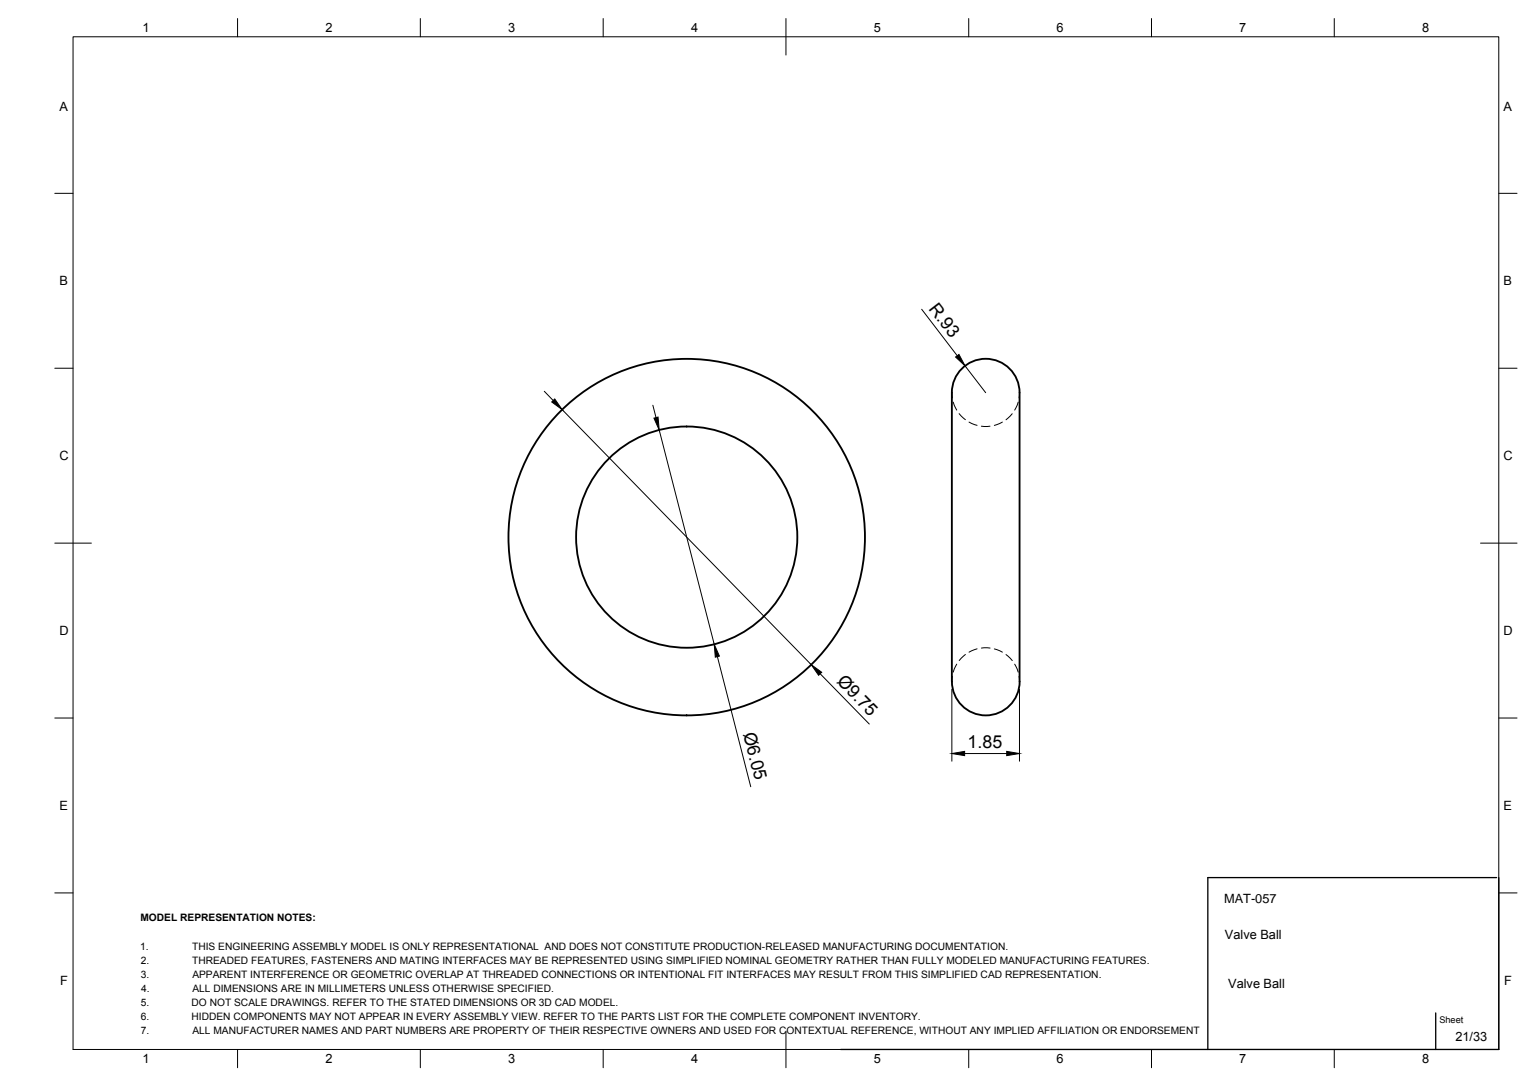
ISO-10303-21;
HEADER;
/* Generated by software containing ST-Developer
 * from STEP Tools, Inc. (www.steptools.com) 
 */

FILE_DESCRIPTION(
/* description */ ('STEP AP214', 'CAx-IF Rec.Pracs.---Representation and Presentation of Product Manufa
cturing Information (PMI)---4.0---2014-10-13'),
/* implementation_level */ '2;1');

FILE_NAME(
/* name */ 'Valve Ball.step',
/* time_stamp */ '2026-10-28T23:34:22+01:00',
/* author */ (''),
/* organization */ (''),
/* preprocessor_version */ 'ST-DEVELOPER v20.2',
/* originating_system */ 'Autodesk Translation Framework v15.17.0.0',
/* authorisation */ '');

FILE_SCHEMA (('AP242_MANAGED_MODEL_BASED_3D_ENGINEERING_MIM_LF { 1 0 10303 442 2 1 4 }'));
ENDSEC;

DATA;
#10=MECHANICAL_DESIGN_GEOMETRIC_PRESENTATION_REPRESENTATION('',(#262),#27807);
#216=SHAPE_REPRESENTATION_RELATIONSHIP('SRR','None',#27913,#238);
#238=ADVANCED_BREP_SHAPE_REPRESENTATION('',(#291),#27793);
#262=STYLED_ITEM('',(#28063),#291);
#291=MANIFOLD_SOLID_BREP('Body1',#12038);
#831=TOROIDAL_SURFACE('',#13209,3.95,0.925000000000001);
#1675=FACE_OUTER_BOUND('',#2451,.T.);
#2451=EDGE_LOOP('',(#9991,#9992,#9993,#9994));
#4811=CIRCLE('',#13210,0.925000000000001);
#4812=CIRCLE('',#13211,3.02500000000001);
#5724=VERTEX_POINT('',#21297);
#7208=EDGE_CURVE('',#5724,#5724,#4811,.T.);
#7209=EDGE_CURVE('',#5724,#5724,#4812,.T.);
#9991=ORIENTED_EDGE('',*,*,#7208,.F.);
#9992=ORIENTED_EDGE('',*,*,#7209,.T.);
#9993=ORIENTED_EDGE('',*,*,#7208,.T.);
#9994=ORIENTED_EDGE('',*,*,#7209,.F.);
#11757=ADVANCED_FACE('',(#1675),#831,.T.);
#12038=CLOSED_SHELL('',(#11757));
#13208=AXIS2_PLACEMENT_3D('',#21295,#16078,#16079);
#13209=AXIS2_PLACEMENT_3D('',#21296,#16080,#16081);
#13210=AXIS2_PLACEMENT_3D('',#21298,#16082,#16083);
#13211=AXIS2_PLACEMENT_3D('',#21299,#16084,#16085);
#16078=DIRECTION('axis',(0.,0.,1.));
#16079=DIRECTION('refdir',(1.,0.,0.));
#16080=DIRECTION('center_axis',(-0.224684645967588,-0.974431531646231,-6.6078080723141E-17));
#16081=DIRECTION('ref_axis',(-0.893873580715706,0.206109575173111,-0.398131717802591));
#16082=DIRECTION('center_axis',(-0.38795209957532,0.0894540840629421,0.917328259283208));
#16083=DIRECTION('ref_axis',(0.893873580715707,-0.206109575173114,0.398131717802587));
#16084=DIRECTION('center_axis',(0.224684645967588,0.974431531646231,6.6078080723141E-17));
#16085=DIRECTION('ref_axis',(-0.893873580715706,0.206109575173111,-0.39813171780259));
#21295=CARTESIAN_POINT('',(0.,0.,0.));
#21296=CARTESIAN_POINT('Origin',(262.314173983718,112.124344754868,260.573593133705));
#21297=CARTESIAN_POINT('',(265.018141565383,111.50086328997,261.777941580057));
#21298=CARTESIAN_POINT('Origin',(265.844974627545,111.310211932935,262.146213419025));
#21299=CARTESIAN_POINT('Origin',(262.314173983718,112.124344754868,260.573593133705));
#27764=UNCERTAINTY_MEASURE_WITH_UNIT(LENGTH_MEASURE(0.01),#27808,
'DISTANCE_ACCURACY_VALUE',
'Maximum model space distance between geometric entities at asserted c
onnectivities');
#27778=UNCERTAINTY_MEASURE_WITH_UNIT(LENGTH_MEASURE(0.01),#27808,
'DISTANCE_ACCURACY_VALUE',
'Maximum model space distance between geometric entities at asserted c
onnectivities');
#27793=(
GEOMETRIC_REPRESENTATION_CONTEXT(3)
GLOBAL_UNCERTAINTY_ASSIGNED_CONTEXT((#27764))
GLOBAL_UNIT_ASSIGNED_CONTEXT((#27808,#27810,#27811))
REPRESENTATION_CONTEXT('','3D')
);
#27807=(
GEOMETRIC_REPRESENTATION_CONTEXT(3)
GLOBAL_UNCERTAINTY_ASSIGNED_CONTEXT((#27778))
GLOBAL_UNIT_ASSIGNED_CONTEXT((#27808,#27810,#27811))
REPRESENTATION_CONTEXT('','3D')
);
#27808=(
LENGTH_UNIT()
NAMED_UNIT(*)
SI_UNIT(.MILLI.,.METRE.)
);
#27810=(
NAMED_UNIT(*)
PLANE_ANGLE_UNIT()
SI_UNIT($,.RADIAN.)
);
#27811=(
NAMED_UNIT(*)
SI_UNIT($,.STERADIAN.)
SOLID_ANGLE_UNIT()
);
#27826=SHAPE_DEFINITION_REPRESENTATION(#27859,#27913);
#27859=PRODUCT_DEFINITION_SHAPE('',$,#27942);
#27913=SHAPE_REPRESENTATION('',(#13208),#27793);
#27927=PRODUCT_DEFINITION_CONTEXT('part definition',#28013,'design');
#27942=PRODUCT_DEFINITION('Valve Ball','Valve Ball',#27970,#27927);
#27970=PRODUCT_DEFINITION_FORMATION('',$,#28029);
#28013=APPLICATION_CONTEXT('Managed model based 3d engineering');
#28014=PRODUCT_CONTEXT('part definition',#28013,'mechanical');
#28029=PRODUCT('Valve Ball','Valve Ball',$,(#28014));
#28057=COLOUR_RGB('Light Blue',0.38,0.62,0.78);
#28058=FILL_AREA_STYLE_COLOUR('',#28057);
#28059=FILL_AREA_STYLE('',(#28058));
#28060=SURFACE_STYLE_FILL_AREA(#28059);
#28061=SURFACE_SIDE_STYLE('',(#28060));
#28062=SURFACE_STYLE_USAGE(.BOTH.,#28061);
#28063=PRESENTATION_STYLE_ASSIGNMENT((#28062));
ENDSEC;
END-ISO-10303-21;
